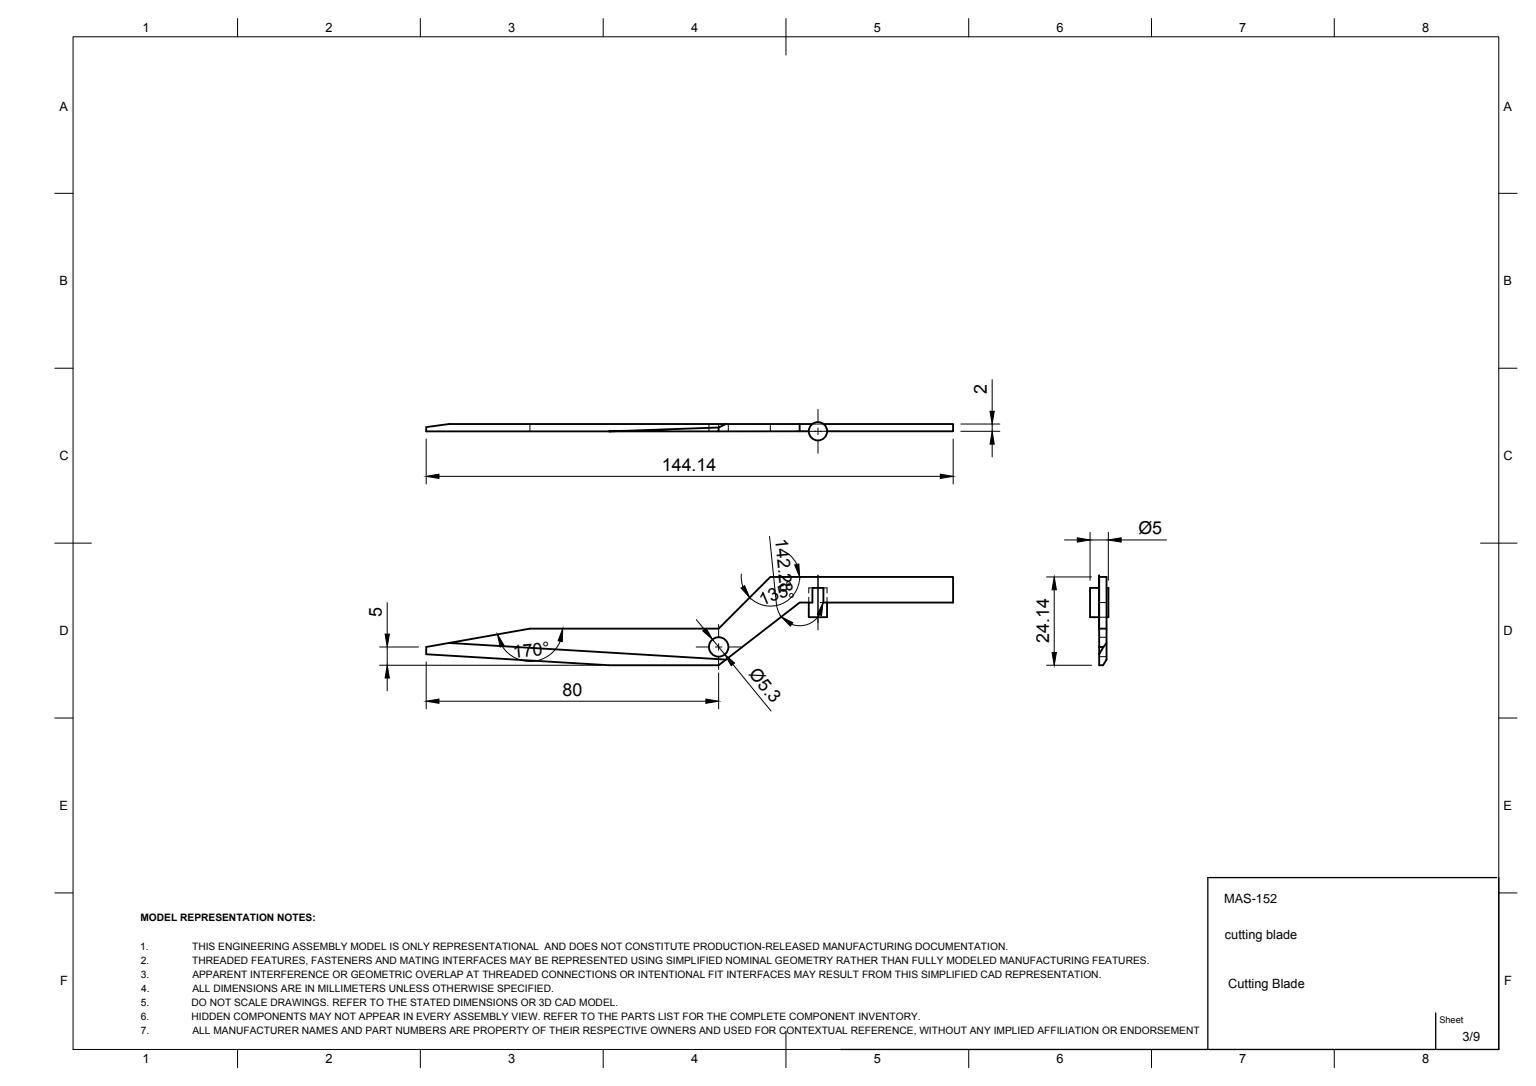
ISO-10303-21;
HEADER;
/* Generated by software containing ST-Developer
 * from STEP Tools, Inc. (www.steptools.com) 
 */

FILE_DESCRIPTION(
/* description */ ('STEP AP214'),
/* implementation_level */ '2;1');

FILE_NAME(
/* name */ 'Cutting Blade.step',
/* time_stamp */ '2026-11-04T19:18:53-08:00',
/* author */ (''),
/* organization */ (''),
/* preprocessor_version */ 'ST-DEVELOPER v20.2',
/* originating_system */ 'Autodesk Translation Framework v15.17.0.0',
/* authorisation */ '');

FILE_SCHEMA (('AUTOMOTIVE_DESIGN { 1 0 10303 214 3 1 1 }'));
ENDSEC;

DATA;
#10=MECHANICAL_DESIGN_GEOMETRIC_PRESENTATION_REPRESENTATION('',(#81),#5942);
#67=SHAPE_REPRESENTATION_RELATIONSHIP('SRR','None',#5978,#74);
#74=ADVANCED_BREP_SHAPE_REPRESENTATION('',(#88),#5938);
#81=STYLED_ITEM('',(#6022),#88);
#88=MANIFOLD_SOLID_BREP('Body1',#928);
#94=FACE_BOUND('',#217,.T.);
#95=FACE_BOUND('',#219,.T.);
#106=PLANE('',#1051);
#107=PLANE('',#1052);
#108=PLANE('',#1053);
#109=PLANE('',#1054);
#110=PLANE('',#1055);
#111=PLANE('',#1056);
#112=PLANE('',#1057);
#113=PLANE('',#1058);
#114=PLANE('',#1059);
#115=PLANE('',#1060);
#116=PLANE('',#1061);
#117=PLANE('',#1062);
#118=PLANE('',#1063);
#119=PLANE('',#1064);
#120=PLANE('',#1065);
#121=PLANE('',#1066);
#154=FACE_OUTER_BOUND('',#210,.T.);
#155=FACE_OUTER_BOUND('',#211,.T.);
#156=FACE_OUTER_BOUND('',#212,.T.);
#157=FACE_OUTER_BOUND('',#213,.T.);
#158=FACE_OUTER_BOUND('',#214,.T.);
#159=FACE_OUTER_BOUND('',#215,.T.);
#160=FACE_OUTER_BOUND('',#216,.T.);
#161=FACE_OUTER_BOUND('',#218,.T.);
#162=FACE_OUTER_BOUND('',#220,.T.);
#163=FACE_OUTER_BOUND('',#221,.T.);
#164=FACE_OUTER_BOUND('',#222,.T.);
#165=FACE_OUTER_BOUND('',#223,.T.);
#166=FACE_OUTER_BOUND('',#224,.T.);
#167=FACE_OUTER_BOUND('',#225,.T.);
#168=FACE_OUTER_BOUND('',#226,.T.);
#169=FACE_OUTER_BOUND('',#227,.T.);
#170=FACE_OUTER_BOUND('',#228,.T.);
#171=FACE_OUTER_BOUND('',#229,.T.);
#210=EDGE_LOOP('',(#682,#683,#684,#685));
#211=EDGE_LOOP('',(#686,#687,#688,#689,#690,#691,#692,#693,#694,#695,#696,
#697));
#212=EDGE_LOOP('',(#698,#699,#700,#701));
#213=EDGE_LOOP('',(#702,#703,#704,#705));
#214=EDGE_LOOP('',(#706,#707,#708));
#215=EDGE_LOOP('',(#709,#710,#711));
#216=EDGE_LOOP('',(#712,#713,#714,#715,#716,#717,#718,#719,#720,#721,#722,
#723));
#217=EDGE_LOOP('',(#724));
#218=EDGE_LOOP('',(#725,#726,#727,#728,#729,#730,#731,#732,#733,#734,#735,
#736,#737,#738));
#219=EDGE_LOOP('',(#739));
#220=EDGE_LOOP('',(#740,#741,#742,#743,#744));
#221=EDGE_LOOP('',(#745,#746,#747,#748));
#222=EDGE_LOOP('',(#749,#750,#751,#752));
#223=EDGE_LOOP('',(#753,#754,#755,#756));
#224=EDGE_LOOP('',(#757,#758,#759,#760));
#225=EDGE_LOOP('',(#761,#762,#763,#764,#765));
#226=EDGE_LOOP('',(#766,#767,#768,#769,#770,#771));
#227=EDGE_LOOP('',(#772,#773));
#228=EDGE_LOOP('',(#774));
#229=EDGE_LOOP('',(#775,#776,#777));
#260=LINE('',#5725,#338);
#261=LINE('',#5731,#339);
#262=LINE('',#5735,#340);
#263=LINE('',#5739,#341);
#264=LINE('',#5743,#342);
#265=LINE('',#5747,#343);
#266=LINE('',#5751,#344);
#267=LINE('',#5753,#345);
#268=LINE('',#5754,#346);
#269=LINE('',#5758,#347);
#270=LINE('',#5760,#348);
#271=LINE('',#5762,#349);
#272=LINE('',#5763,#350);
#273=LINE('',#5767,#351);
#274=LINE('',#5769,#352);
#275=LINE('',#5770,#353);
#276=LINE('',#5774,#354);
#277=LINE('',#5776,#355);
#278=LINE('',#5777,#356);
#279=LINE('',#5779,#357);
#280=LINE('',#5781,#358);
#281=LINE('',#5783,#359);
#282=LINE('',#5784,#360);
#283=LINE('',#5786,#361);
#284=LINE('',#5788,#362);
#285=LINE('',#5790,#363);
#286=LINE('',#5791,#364);
#287=LINE('',#5793,#365);
#288=LINE('',#5795,#366);
#289=LINE('',#5796,#367);
#290=LINE('',#5797,#368);
#291=LINE('',#5798,#369);
#292=LINE('',#5800,#370);
#293=LINE('',#5802,#371);
#294=LINE('',#5803,#372);
#295=LINE('',#5805,#373);
#296=LINE('',#5806,#374);
#297=LINE('',#5808,#375);
#298=LINE('',#5810,#376);
#299=LINE('',#5814,#377);
#338=VECTOR('',#1181,2.65);
#339=VECTOR('',#1188,2.5);
#340=VECTOR('',#1191,1000.);
#341=VECTOR('',#1194,1000.);
#342=VECTOR('',#1197,1000.);
#343=VECTOR('',#1200,1000.);
#344=VECTOR('',#1205,1000.);
#345=VECTOR('',#1206,1000.);
#346=VECTOR('',#1207,1000.);
#347=VECTOR('',#1210,1000.);
#348=VECTOR('',#1211,1000.);
#349=VECTOR('',#1212,1000.);
#350=VECTOR('',#1213,1000.);
#351=VECTOR('',#1216,1000.);
#352=VECTOR('',#1217,1000.);
#353=VECTOR('',#1218,1000.);
#354=VECTOR('',#1221,1000.);
#355=VECTOR('',#1222,1000.);
#356=VECTOR('',#1223,1000.);
#357=VECTOR('',#1226,1000.);
#358=VECTOR('',#1227,1000.);
#359=VECTOR('',#1228,1000.);
#360=VECTOR('',#1229,1000.);
#361=VECTOR('',#1230,1000.);
#362=VECTOR('',#1231,1000.);
#363=VECTOR('',#1232,1000.);
#364=VECTOR('',#1233,1000.);
#365=VECTOR('',#1236,1000.);
#366=VECTOR('',#1237,1000.);
#367=VECTOR('',#1238,1000.);
#368=VECTOR('',#1239,1000.);
#369=VECTOR('',#1240,1000.);
#370=VECTOR('',#1241,1000.);
#371=VECTOR('',#1242,1000.);
#372=VECTOR('',#1243,1000.);
#373=VECTOR('',#1246,1000.);
#374=VECTOR('',#1247,1000.);
#375=VECTOR('',#1250,1000.);
#376=VECTOR('',#1253,1000.);
#377=VECTOR('',#1260,1000.);
#428=CIRCLE('',#1042,2.65);
#429=CIRCLE('',#1043,2.65);
#430=CIRCLE('',#1045,2.5);
#431=CIRCLE('',#1046,2.5);
#432=CIRCLE('',#1047,2.5);
#433=CIRCLE('',#1048,2.5);
#434=CIRCLE('',#1049,2.5);
#435=CIRCLE('',#1050,2.5);
#460=VERTEX_POINT('',#5722);
#461=VERTEX_POINT('',#5724);
#462=VERTEX_POINT('',#5728);
#463=VERTEX_POINT('',#5730);
#464=VERTEX_POINT('',#5732);
#465=VERTEX_POINT('',#5734);
#466=VERTEX_POINT('',#5736);
#467=VERTEX_POINT('',#5738);
#468=VERTEX_POINT('',#5740);
#469=VERTEX_POINT('',#5742);
#470=VERTEX_POINT('',#5744);
#471=VERTEX_POINT('',#5746);
#472=VERTEX_POINT('',#5750);
#473=VERTEX_POINT('',#5752);
#474=VERTEX_POINT('',#5756);
#475=VERTEX_POINT('',#5757);
#476=VERTEX_POINT('',#5759);
#477=VERTEX_POINT('',#5761);
#478=VERTEX_POINT('',#5765);
#479=VERTEX_POINT('',#5766);
#480=VERTEX_POINT('',#5768);
#481=VERTEX_POINT('',#5772);
#482=VERTEX_POINT('',#5773);
#483=VERTEX_POINT('',#5775);
#484=VERTEX_POINT('',#5780);
#485=VERTEX_POINT('',#5782);
#486=VERTEX_POINT('',#5785);
#487=VERTEX_POINT('',#5787);
#488=VERTEX_POINT('',#5789);
#489=VERTEX_POINT('',#5794);
#490=VERTEX_POINT('',#5799);
#491=VERTEX_POINT('',#5801);
#544=EDGE_CURVE('',#460,#460,#428,.T.);
#545=EDGE_CURVE('',#460,#461,#260,.T.);
#546=EDGE_CURVE('',#461,#461,#429,.T.);
#547=EDGE_CURVE('',#462,#462,#430,.T.);
#548=EDGE_CURVE('',#462,#463,#261,.T.);
#549=EDGE_CURVE('',#463,#464,#431,.T.);
#550=EDGE_CURVE('',#464,#465,#262,.T.);
#551=EDGE_CURVE('',#465,#466,#432,.T.);
#552=EDGE_CURVE('',#467,#466,#263,.T.);
#553=EDGE_CURVE('',#467,#468,#433,.T.);
#554=EDGE_CURVE('',#469,#468,#264,.T.);
#555=EDGE_CURVE('',#469,#470,#434,.T.);
#556=EDGE_CURVE('',#470,#471,#265,.T.);
#557=EDGE_CURVE('',#471,#463,#435,.T.);
#558=EDGE_CURVE('',#465,#472,#266,.T.);
#559=EDGE_CURVE('',#472,#473,#267,.T.);
#560=EDGE_CURVE('',#466,#473,#268,.T.);
#561=EDGE_CURVE('',#474,#475,#269,.T.);
#562=EDGE_CURVE('',#475,#476,#270,.T.);
#563=EDGE_CURVE('',#477,#476,#271,.T.);
#564=EDGE_CURVE('',#477,#474,#272,.T.);
#565=EDGE_CURVE('',#478,#479,#273,.T.);
#566=EDGE_CURVE('',#478,#480,#274,.T.);
#567=EDGE_CURVE('',#480,#479,#275,.T.);
#568=EDGE_CURVE('',#481,#482,#276,.T.);
#569=EDGE_CURVE('',#481,#483,#277,.T.);
#570=EDGE_CURVE('',#482,#483,#278,.T.);
#571=EDGE_CURVE('',#467,#468,#279,.T.);
#572=EDGE_CURVE('',#473,#484,#280,.T.);
#573=EDGE_CURVE('',#484,#485,#281,.T.);
#574=EDGE_CURVE('',#485,#477,#282,.T.);
#575=EDGE_CURVE('',#476,#486,#283,.T.);
#576=EDGE_CURVE('',#486,#487,#284,.T.);
#577=EDGE_CURVE('',#487,#488,#285,.T.);
#578=EDGE_CURVE('',#488,#469,#286,.T.);
#579=EDGE_CURVE('',#464,#471,#287,.T.);
#580=EDGE_CURVE('',#489,#470,#288,.T.);
#581=EDGE_CURVE('',#482,#489,#289,.T.);
#582=EDGE_CURVE('',#483,#478,#290,.T.);
#583=EDGE_CURVE('',#479,#475,#291,.T.);
#584=EDGE_CURVE('',#490,#474,#292,.T.);
#585=EDGE_CURVE('',#491,#490,#293,.T.);
#586=EDGE_CURVE('',#472,#491,#294,.T.);
#587=EDGE_CURVE('',#487,#481,#295,.T.);
#588=EDGE_CURVE('',#489,#488,#296,.T.);
#589=EDGE_CURVE('',#490,#485,#297,.T.);
#590=EDGE_CURVE('',#491,#484,#298,.T.);
#591=EDGE_CURVE('',#480,#486,#299,.T.);
#682=ORIENTED_EDGE('',*,*,#544,.T.);
#683=ORIENTED_EDGE('',*,*,#545,.T.);
#684=ORIENTED_EDGE('',*,*,#546,.T.);
#685=ORIENTED_EDGE('',*,*,#545,.F.);
#686=ORIENTED_EDGE('',*,*,#547,.F.);
#687=ORIENTED_EDGE('',*,*,#548,.T.);
#688=ORIENTED_EDGE('',*,*,#549,.T.);
#689=ORIENTED_EDGE('',*,*,#550,.T.);
#690=ORIENTED_EDGE('',*,*,#551,.T.);
#691=ORIENTED_EDGE('',*,*,#552,.F.);
#692=ORIENTED_EDGE('',*,*,#553,.T.);
#693=ORIENTED_EDGE('',*,*,#554,.F.);
#694=ORIENTED_EDGE('',*,*,#555,.T.);
#695=ORIENTED_EDGE('',*,*,#556,.T.);
#696=ORIENTED_EDGE('',*,*,#557,.T.);
#697=ORIENTED_EDGE('',*,*,#548,.F.);
#698=ORIENTED_EDGE('',*,*,#551,.F.);
#699=ORIENTED_EDGE('',*,*,#558,.T.);
#700=ORIENTED_EDGE('',*,*,#559,.T.);
#701=ORIENTED_EDGE('',*,*,#560,.F.);
#702=ORIENTED_EDGE('',*,*,#561,.T.);
#703=ORIENTED_EDGE('',*,*,#562,.T.);
#704=ORIENTED_EDGE('',*,*,#563,.F.);
#705=ORIENTED_EDGE('',*,*,#564,.T.);
#706=ORIENTED_EDGE('',*,*,#565,.F.);
#707=ORIENTED_EDGE('',*,*,#566,.T.);
#708=ORIENTED_EDGE('',*,*,#567,.T.);
#709=ORIENTED_EDGE('',*,*,#568,.F.);
#710=ORIENTED_EDGE('',*,*,#569,.T.);
#711=ORIENTED_EDGE('',*,*,#570,.F.);
#712=ORIENTED_EDGE('',*,*,#571,.F.);
#713=ORIENTED_EDGE('',*,*,#552,.T.);
#714=ORIENTED_EDGE('',*,*,#560,.T.);
#715=ORIENTED_EDGE('',*,*,#572,.T.);
#716=ORIENTED_EDGE('',*,*,#573,.T.);
#717=ORIENTED_EDGE('',*,*,#574,.T.);
#718=ORIENTED_EDGE('',*,*,#563,.T.);
#719=ORIENTED_EDGE('',*,*,#575,.T.);
#720=ORIENTED_EDGE('',*,*,#576,.T.);
#721=ORIENTED_EDGE('',*,*,#577,.T.);
#722=ORIENTED_EDGE('',*,*,#578,.T.);
#723=ORIENTED_EDGE('',*,*,#554,.T.);
#724=ORIENTED_EDGE('',*,*,#546,.F.);
#725=ORIENTED_EDGE('',*,*,#550,.F.);
#726=ORIENTED_EDGE('',*,*,#579,.T.);
#727=ORIENTED_EDGE('',*,*,#556,.F.);
#728=ORIENTED_EDGE('',*,*,#580,.F.);
#729=ORIENTED_EDGE('',*,*,#581,.F.);
#730=ORIENTED_EDGE('',*,*,#570,.T.);
#731=ORIENTED_EDGE('',*,*,#582,.T.);
#732=ORIENTED_EDGE('',*,*,#565,.T.);
#733=ORIENTED_EDGE('',*,*,#583,.T.);
#734=ORIENTED_EDGE('',*,*,#561,.F.);
#735=ORIENTED_EDGE('',*,*,#584,.F.);
#736=ORIENTED_EDGE('',*,*,#585,.F.);
#737=ORIENTED_EDGE('',*,*,#586,.F.);
#738=ORIENTED_EDGE('',*,*,#558,.F.);
#739=ORIENTED_EDGE('',*,*,#544,.F.);
#740=ORIENTED_EDGE('',*,*,#577,.F.);
#741=ORIENTED_EDGE('',*,*,#587,.T.);
#742=ORIENTED_EDGE('',*,*,#568,.T.);
#743=ORIENTED_EDGE('',*,*,#581,.T.);
#744=ORIENTED_EDGE('',*,*,#588,.T.);
#745=ORIENTED_EDGE('',*,*,#574,.F.);
#746=ORIENTED_EDGE('',*,*,#589,.F.);
#747=ORIENTED_EDGE('',*,*,#584,.T.);
#748=ORIENTED_EDGE('',*,*,#564,.F.);
#749=ORIENTED_EDGE('',*,*,#573,.F.);
#750=ORIENTED_EDGE('',*,*,#590,.F.);
#751=ORIENTED_EDGE('',*,*,#585,.T.);
#752=ORIENTED_EDGE('',*,*,#589,.T.);
#753=ORIENTED_EDGE('',*,*,#572,.F.);
#754=ORIENTED_EDGE('',*,*,#559,.F.);
#755=ORIENTED_EDGE('',*,*,#586,.T.);
#756=ORIENTED_EDGE('',*,*,#590,.T.);
#757=ORIENTED_EDGE('',*,*,#555,.F.);
#758=ORIENTED_EDGE('',*,*,#578,.F.);
#759=ORIENTED_EDGE('',*,*,#588,.F.);
#760=ORIENTED_EDGE('',*,*,#580,.T.);
#761=ORIENTED_EDGE('',*,*,#567,.F.);
#762=ORIENTED_EDGE('',*,*,#591,.T.);
#763=ORIENTED_EDGE('',*,*,#575,.F.);
#764=ORIENTED_EDGE('',*,*,#562,.F.);
#765=ORIENTED_EDGE('',*,*,#583,.F.);
#766=ORIENTED_EDGE('',*,*,#566,.F.);
#767=ORIENTED_EDGE('',*,*,#582,.F.);
#768=ORIENTED_EDGE('',*,*,#569,.F.);
#769=ORIENTED_EDGE('',*,*,#587,.F.);
#770=ORIENTED_EDGE('',*,*,#576,.F.);
#771=ORIENTED_EDGE('',*,*,#591,.F.);
#772=ORIENTED_EDGE('',*,*,#553,.F.);
#773=ORIENTED_EDGE('',*,*,#571,.T.);
#774=ORIENTED_EDGE('',*,*,#547,.T.);
#775=ORIENTED_EDGE('',*,*,#579,.F.);
#776=ORIENTED_EDGE('',*,*,#549,.F.);
#777=ORIENTED_EDGE('',*,*,#557,.F.);
#865=CYLINDRICAL_SURFACE('',#1041,2.65);
#866=CYLINDRICAL_SURFACE('',#1044,2.5);
#885=ADVANCED_FACE('',(#154),#865,.F.);
#886=ADVANCED_FACE('',(#155),#866,.T.);
#887=ADVANCED_FACE('',(#156),#106,.T.);
#888=ADVANCED_FACE('',(#157),#107,.F.);
#889=ADVANCED_FACE('',(#158),#108,.T.);
#890=ADVANCED_FACE('',(#159),#109,.T.);
#891=ADVANCED_FACE('',(#160,#94),#110,.F.);
#892=ADVANCED_FACE('',(#161,#95),#111,.T.);
#893=ADVANCED_FACE('',(#162),#112,.T.);
#894=ADVANCED_FACE('',(#163),#113,.T.);
#895=ADVANCED_FACE('',(#164),#114,.T.);
#896=ADVANCED_FACE('',(#165),#115,.T.);
#897=ADVANCED_FACE('',(#166),#116,.T.);
#898=ADVANCED_FACE('',(#167),#117,.T.);
#899=ADVANCED_FACE('',(#168),#118,.F.);
#900=ADVANCED_FACE('',(#169),#119,.F.);
#901=ADVANCED_FACE('',(#170),#120,.T.);
#902=ADVANCED_FACE('',(#171),#121,.F.);
#928=CLOSED_SHELL('',(#885,#886,#887,#888,#889,#890,#891,#892,#893,#894,
#895,#896,#897,#898,#899,#900,#901,#902));
#1040=AXIS2_PLACEMENT_3D('',#5720,#1175,#1176);
#1041=AXIS2_PLACEMENT_3D('',#5721,#1177,#1178);
#1042=AXIS2_PLACEMENT_3D('',#5723,#1179,#1180);
#1043=AXIS2_PLACEMENT_3D('',#5726,#1182,#1183);
#1044=AXIS2_PLACEMENT_3D('',#5727,#1184,#1185);
#1045=AXIS2_PLACEMENT_3D('',#5729,#1186,#1187);
#1046=AXIS2_PLACEMENT_3D('',#5733,#1189,#1190);
#1047=AXIS2_PLACEMENT_3D('',#5737,#1192,#1193);
#1048=AXIS2_PLACEMENT_3D('',#5741,#1195,#1196);
#1049=AXIS2_PLACEMENT_3D('',#5745,#1198,#1199);
#1050=AXIS2_PLACEMENT_3D('',#5748,#1201,#1202);
#1051=AXIS2_PLACEMENT_3D('',#5749,#1203,#1204);
#1052=AXIS2_PLACEMENT_3D('',#5755,#1208,#1209);
#1053=AXIS2_PLACEMENT_3D('',#5764,#1214,#1215);
#1054=AXIS2_PLACEMENT_3D('',#5771,#1219,#1220);
#1055=AXIS2_PLACEMENT_3D('',#5778,#1224,#1225);
#1056=AXIS2_PLACEMENT_3D('',#5792,#1234,#1235);
#1057=AXIS2_PLACEMENT_3D('',#5804,#1244,#1245);
#1058=AXIS2_PLACEMENT_3D('',#5807,#1248,#1249);
#1059=AXIS2_PLACEMENT_3D('',#5809,#1251,#1252);
#1060=AXIS2_PLACEMENT_3D('',#5811,#1254,#1255);
#1061=AXIS2_PLACEMENT_3D('',#5812,#1256,#1257);
#1062=AXIS2_PLACEMENT_3D('',#5813,#1258,#1259);
#1063=AXIS2_PLACEMENT_3D('',#5815,#1261,#1262);
#1064=AXIS2_PLACEMENT_3D('',#5816,#1263,#1264);
#1065=AXIS2_PLACEMENT_3D('',#5817,#1265,#1266);
#1066=AXIS2_PLACEMENT_3D('',#5818,#1267,#1268);
#1175=DIRECTION('axis',(0.,0.,1.));
#1176=DIRECTION('refdir',(1.,0.,0.));
#1177=DIRECTION('center_axis',(0.,0.,1.));
#1178=DIRECTION('ref_axis',(1.,0.,0.));
#1179=DIRECTION('center_axis',(0.,0.,-1.));
#1180=DIRECTION('ref_axis',(-1.,0.,0.));
#1181=DIRECTION('',(0.,0.,1.));
#1182=DIRECTION('center_axis',(0.,0.,1.));
#1183=DIRECTION('ref_axis',(1.,0.,0.));
#1184=DIRECTION('center_axis',(-1.,0.,0.));
#1185=DIRECTION('ref_axis',(0.,0.,1.));
#1186=DIRECTION('center_axis',(-1.,0.,0.));
#1187=DIRECTION('ref_axis',(0.,0.,1.));
#1188=DIRECTION('',(1.,0.,0.));
#1189=DIRECTION('center_axis',(-1.,0.,0.));
#1190=DIRECTION('ref_axis',(0.,0.,1.));
#1191=DIRECTION('',(-1.,0.,0.));
#1192=DIRECTION('center_axis',(-1.,-1.51313062618285E-16,0.));
#1193=DIRECTION('ref_axis',(1.51313062618285E-16,-1.,0.));
#1194=DIRECTION('',(-1.,0.,0.));
#1195=DIRECTION('center_axis',(-1.,0.,0.));
#1196=DIRECTION('ref_axis',(0.,0.,1.));
#1197=DIRECTION('',(1.,0.,0.));
#1198=DIRECTION('center_axis',(-1.,-1.51313062618285E-16,0.));
#1199=DIRECTION('ref_axis',(1.51313062618285E-16,-1.,0.));
#1200=DIRECTION('',(1.,0.,0.));
#1201=DIRECTION('center_axis',(-1.,0.,0.));
#1202=DIRECTION('ref_axis',(0.,0.,1.));
#1203=DIRECTION('center_axis',(-1.,-1.51313062618285E-16,0.));
#1204=DIRECTION('ref_axis',(1.51313062618285E-16,-1.,0.));
#1205=DIRECTION('',(1.51313062618285E-16,-1.,0.));
#1206=DIRECTION('',(0.,0.,1.));
#1207=DIRECTION('',(1.51313062618285E-16,-1.,0.));
#1208=DIRECTION('center_axis',(-1.,0.,0.));
#1209=DIRECTION('ref_axis',(0.,0.,1.));
#1210=DIRECTION('',(0.,1.,0.));
#1211=DIRECTION('',(0.,0.,1.));
#1212=DIRECTION('',(0.,1.,0.));
#1213=DIRECTION('',(0.,0.,-1.));
#1214=DIRECTION('center_axis',(0.,1.,0.));
#1215=DIRECTION('ref_axis',(0.,0.,1.));
#1216=DIRECTION('',(1.,0.,0.));
#1217=DIRECTION('',(0.866413978654257,0.,0.499326363806779));
#1218=DIRECTION('',(0.,0.,-1.));
#1219=DIRECTION('center_axis',(-1.,0.,0.));
#1220=DIRECTION('ref_axis',(0.,0.,1.));
#1221=DIRECTION('',(0.,0.,-1.));
#1222=DIRECTION('',(0.,0.999402687851137,-0.0345581758188068));
#1223=DIRECTION('',(0.,1.,0.));
#1224=DIRECTION('center_axis',(0.,0.,-1.));
#1225=DIRECTION('ref_axis',(-1.,0.,0.));
#1226=DIRECTION('',(0.,1.,0.));
#1227=DIRECTION('',(1.,0.,0.));
#1228=DIRECTION('',(-6.93889390390723E-17,1.,0.));
#1229=DIRECTION('',(-0.707106781186544,0.707106781186551,0.));
#1230=DIRECTION('',(-0.17364817766693,0.984807753012208,0.));
#1231=DIRECTION('',(-0.0598922907279467,-0.998204845465779,0.));
#1232=DIRECTION('',(0.611809881784581,-0.791004847362351,0.));
#1233=DIRECTION('',(1.51313062618285E-16,-1.,0.));
#1234=DIRECTION('center_axis',(0.,0.,-1.));
#1235=DIRECTION('ref_axis',(-1.,0.,0.));
#1236=DIRECTION('',(0.,1.,0.));
#1237=DIRECTION('',(1.51313062618285E-16,-1.,0.));
#1238=DIRECTION('',(0.611809881784581,-0.791004847362351,0.));
#1239=DIRECTION('',(0.0598922907279467,0.998204845465779,0.));
#1240=DIRECTION('',(0.17364817766693,-0.984807753012208,0.));
#1241=DIRECTION('',(-0.707106781186544,0.707106781186551,0.));
#1242=DIRECTION('',(-6.93889390390723E-17,1.,0.));
#1243=DIRECTION('',(1.,0.,0.));
#1244=DIRECTION('center_axis',(-0.791004847362351,-0.611809881784581,0.));
#1245=DIRECTION('ref_axis',(0.611809881784581,-0.791004847362351,0.));
#1246=DIRECTION('',(-0.571919987099744,0.739431473025142,-0.355174077116697));
#1247=DIRECTION('',(0.,0.,1.));
#1248=DIRECTION('center_axis',(0.707106781186551,0.707106781186544,0.));
#1249=DIRECTION('ref_axis',(-0.707106781186544,0.707106781186551,0.));
#1250=DIRECTION('',(0.,0.,1.));
#1251=DIRECTION('center_axis',(1.,6.93889390390723E-17,0.));
#1252=DIRECTION('ref_axis',(-6.93889390390723E-17,1.,0.));
#1253=DIRECTION('',(0.,0.,1.));
#1254=DIRECTION('center_axis',(0.,-1.,0.));
#1255=DIRECTION('ref_axis',(0.,0.,-1.));
#1256=DIRECTION('center_axis',(-1.,-1.51313062618285E-16,0.));
#1257=DIRECTION('ref_axis',(1.51313062618285E-16,-1.,0.));
#1258=DIRECTION('center_axis',(0.984807753012208,0.17364817766693,0.));
#1259=DIRECTION('ref_axis',(0.,0.,1.));
#1260=DIRECTION('',(0.172106918435043,-0.976066837551089,0.132938847820377));
#1261=DIRECTION('center_axis',(0.499102422732889,-0.0299461453639734,-0.866025403784439));
#1262=DIRECTION('ref_axis',(-0.0598922907279467,-0.998204845465779,1.0301470331017E-18));
#1263=DIRECTION('center_axis',(-1.,0.,0.));
#1264=DIRECTION('ref_axis',(0.,0.,1.));
#1265=DIRECTION('center_axis',(-1.,0.,0.));
#1266=DIRECTION('ref_axis',(0.,0.,1.));
#1267=DIRECTION('center_axis',(-1.,0.,0.));
#1268=DIRECTION('ref_axis',(0.,0.,1.));
#5720=CARTESIAN_POINT('',(0.,0.,0.));
#5721=CARTESIAN_POINT('Origin',(0.,0.,2.));
#5722=CARTESIAN_POINT('',(-2.65,-3.24531401774049E-16,0.));
#5723=CARTESIAN_POINT('Origin',(0.,0.,0.));
#5724=CARTESIAN_POINT('',(-2.65,-3.24531401774049E-16,2.));
#5725=CARTESIAN_POINT('',(-2.65,-3.24531401774049E-16,2.));
#5726=CARTESIAN_POINT('Origin',(0.,0.,2.));
#5727=CARTESIAN_POINT('Origin',(16.1421356237309,-27.1629509039023,0.));
#5728=CARTESIAN_POINT('',(8.14213562373088,-27.1629509039023,-2.5));
#5729=CARTESIAN_POINT('Origin',(8.14213562373088,-27.1629509039023,0.));
#5730=CARTESIAN_POINT('',(16.1421356237309,-27.1629509039023,-2.5));
#5731=CARTESIAN_POINT('',(16.1421356237309,-27.1629509039023,-2.5));
#5732=CARTESIAN_POINT('',(16.1421356237309,-29.6629509039023,0.));
#5733=CARTESIAN_POINT('Origin',(16.1421356237309,-27.1629509039023,0.));
#5734=CARTESIAN_POINT('',(12.1421356237309,-29.6629509039023,0.));
#5735=CARTESIAN_POINT('',(16.1421356237309,-29.6629509039023,0.));
#5736=CARTESIAN_POINT('',(12.1421356237309,-28.6629509039023,2.));
#5737=CARTESIAN_POINT('Origin',(12.1421356237309,-27.1629509039023,0.));
#5738=CARTESIAN_POINT('',(16.1421356237309,-28.6629509039023,2.));
#5739=CARTESIAN_POINT('',(16.1421356237309,-28.6629509039023,2.));
#5740=CARTESIAN_POINT('',(16.1421356237309,-25.6629509039023,2.));
#5741=CARTESIAN_POINT('Origin',(16.1421356237309,-27.1629509039023,0.));
#5742=CARTESIAN_POINT('',(12.1421356237309,-25.6629509039023,2.));
#5743=CARTESIAN_POINT('',(16.1421356237309,-25.6629509039023,2.));
#5744=CARTESIAN_POINT('',(12.1421356237309,-24.6629509039023,0.));
#5745=CARTESIAN_POINT('Origin',(12.1421356237309,-27.1629509039023,0.));
#5746=CARTESIAN_POINT('',(16.1421356237309,-24.6629509039023,0.));
#5747=CARTESIAN_POINT('',(16.1421356237309,-24.6629509039023,0.));
#5748=CARTESIAN_POINT('Origin',(16.1421356237309,-27.1629509039023,0.));
#5749=CARTESIAN_POINT('Origin',(12.1421356237309,-18.2842712474619,0.));
#5750=CARTESIAN_POINT('',(12.1421356237309,-64.142135623731,0.));
#5751=CARTESIAN_POINT('',(12.1421356237309,-18.2842712474619,0.));
#5752=CARTESIAN_POINT('',(12.1421356237309,-64.142135623731,2.));
#5753=CARTESIAN_POINT('',(12.1421356237309,-64.142135623731,0.));
#5754=CARTESIAN_POINT('',(12.1421356237309,-18.2842712474619,2.));
#5755=CARTESIAN_POINT('Origin',(5.,0.,2.));
#5756=CARTESIAN_POINT('',(5.,0.,0.));
#5757=CARTESIAN_POINT('',(5.,51.6435909019114,0.));
#5758=CARTESIAN_POINT('',(5.,0.,0.));
#5759=CARTESIAN_POINT('',(5.,51.6435909019114,2.));
#5760=CARTESIAN_POINT('',(5.,51.6435909019114,2.));
#5761=CARTESIAN_POINT('',(5.,0.,2.));
#5762=CARTESIAN_POINT('',(5.,0.,2.));
#5763=CARTESIAN_POINT('',(5.,0.,2.));
#5764=CARTESIAN_POINT('Origin',(-5.,80.,2.));
#5765=CARTESIAN_POINT('',(-2.,80.,0.));
#5766=CARTESIAN_POINT('',(-4.33680868994202E-15,80.,0.));
#5767=CARTESIAN_POINT('',(-5.,80.,0.));
#5768=CARTESIAN_POINT('',(-4.33680868994202E-15,80.,1.15262767247211));
#5769=CARTESIAN_POINT('',(-3.38677286419691,80.,-0.799216389353386));
#5770=CARTESIAN_POINT('',(-4.33680868994202E-15,80.,0.));
#5771=CARTESIAN_POINT('Origin',(-5.,0.,2.));
#5772=CARTESIAN_POINT('',(-5.,0.,1.0373649052249));
#5773=CARTESIAN_POINT('',(-5.,0.,0.));
#5774=CARTESIAN_POINT('',(-5.,0.,2.));
#5775=CARTESIAN_POINT('',(-5.,30.,0.));
#5776=CARTESIAN_POINT('',(-5.,-0.0332470421233885,1.03851454904828));
#5777=CARTESIAN_POINT('',(-5.,0.,0.));
#5778=CARTESIAN_POINT('Origin',(0.,0.,2.));
#5779=CARTESIAN_POINT('',(16.1421356237309,0.,2.));
#5780=CARTESIAN_POINT('',(19.1421356237309,-64.142135623731,2.));
#5781=CARTESIAN_POINT('',(9.14213562373088,-64.142135623731,2.));
#5782=CARTESIAN_POINT('',(19.1421356237309,-14.142135623731,2.));
#5783=CARTESIAN_POINT('',(19.1421356237309,-14.142135623731,2.));
#5784=CARTESIAN_POINT('',(5.,0.,2.));
#5785=CARTESIAN_POINT('',(1.09703553512821,73.7784023141528,2.));
#5786=CARTESIAN_POINT('',(-4.33680868994202E-15,80.,2.));
#5787=CARTESIAN_POINT('',(-3.44991431960659,-2.00409526476049,2.));
#5788=CARTESIAN_POINT('',(-1.54211698258366,29.792527018955,2.));
#5789=CARTESIAN_POINT('',(12.1421356237309,-22.1629509039023,2.));
#5790=CARTESIAN_POINT('',(-5.,0.,2.));
#5791=CARTESIAN_POINT('',(12.1421356237309,-18.2842712474619,2.));
#5792=CARTESIAN_POINT('Origin',(0.,0.,0.));
#5793=CARTESIAN_POINT('',(16.1421356237309,0.,0.));
#5794=CARTESIAN_POINT('',(12.1421356237309,-22.1629509039023,0.));
#5795=CARTESIAN_POINT('',(12.1421356237309,-18.2842712474619,0.));
#5796=CARTESIAN_POINT('',(-5.,0.,0.));
#5797=CARTESIAN_POINT('',(-6.77560781187724,0.406536468712635,0.));
#5798=CARTESIAN_POINT('',(13.6808057330267,2.41229516856365,0.));
#5799=CARTESIAN_POINT('',(19.1421356237309,-14.142135623731,0.));
#5800=CARTESIAN_POINT('',(5.,0.,0.));
#5801=CARTESIAN_POINT('',(19.1421356237309,-64.142135623731,0.));
#5802=CARTESIAN_POINT('',(19.1421356237309,-14.142135623731,0.));
#5803=CARTESIAN_POINT('',(9.14213562373088,-64.142135623731,0.));
#5804=CARTESIAN_POINT('Origin',(-5.,0.,0.));
#5805=CARTESIAN_POINT('',(-5.21072112990534,0.272439919915319,0.906502748749744));
#5806=CARTESIAN_POINT('',(12.1421356237309,-22.1629509039023,0.));
#5807=CARTESIAN_POINT('Origin',(5.,0.,0.));
#5808=CARTESIAN_POINT('',(19.1421356237309,-14.142135623731,0.));
#5809=CARTESIAN_POINT('Origin',(19.1421356237309,-14.142135623731,0.));
#5810=CARTESIAN_POINT('',(19.1421356237309,-64.142135623731,0.));
#5811=CARTESIAN_POINT('Origin',(9.14213562373088,-64.142135623731,0.));
#5812=CARTESIAN_POINT('Origin',(12.1421356237309,-18.2842712474619,0.));
#5813=CARTESIAN_POINT('Origin',(-4.33680868994202E-15,80.,2.));
#5814=CARTESIAN_POINT('',(0.019387620776991,79.8900473387618,1.16760306097774));
#5815=CARTESIAN_POINT('Origin',(-3.3177247944609,0.199063487667654,2.));
#5816=CARTESIAN_POINT('Origin',(16.1421356237309,-27.1629509039023,0.));
#5817=CARTESIAN_POINT('Origin',(8.14213562373088,-27.1629509039023,0.));
#5818=CARTESIAN_POINT('Origin',(16.1421356237309,-27.1629509039023,0.));
#5929=UNCERTAINTY_MEASURE_WITH_UNIT(LENGTH_MEASURE(0.01),#5943,
'DISTANCE_ACCURACY_VALUE',
'Maximum model space distance between geometric entities at asserted c
onnectivities');
#5933=UNCERTAINTY_MEASURE_WITH_UNIT(LENGTH_MEASURE(0.01),#5943,
'DISTANCE_ACCURACY_VALUE',
'Maximum model space distance between geometric entities at asserted c
onnectivities');
#5938=(
GEOMETRIC_REPRESENTATION_CONTEXT(3)
GLOBAL_UNCERTAINTY_ASSIGNED_CONTEXT((#5929))
GLOBAL_UNIT_ASSIGNED_CONTEXT((#5943,#5945,#5946))
REPRESENTATION_CONTEXT('','3D')
);
#5942=(
GEOMETRIC_REPRESENTATION_CONTEXT(3)
GLOBAL_UNCERTAINTY_ASSIGNED_CONTEXT((#5933))
GLOBAL_UNIT_ASSIGNED_CONTEXT((#5943,#5945,#5946))
REPRESENTATION_CONTEXT('','3D')
);
#5943=(
LENGTH_UNIT()
NAMED_UNIT(*)
SI_UNIT(.MILLI.,.METRE.)
);
#5945=(
NAMED_UNIT(*)
PLANE_ANGLE_UNIT()
SI_UNIT($,.RADIAN.)
);
#5946=(
NAMED_UNIT(*)
SI_UNIT($,.STERADIAN.)
SOLID_ANGLE_UNIT()
);
#5951=SHAPE_DEFINITION_REPRESENTATION(#5959,#5978);
#5959=PRODUCT_DEFINITION_SHAPE('',$,#5987);
#5978=SHAPE_REPRESENTATION('',(#1040),#5938);
#5982=PRODUCT_DEFINITION_CONTEXT('part definition',#6008,'design');
#5987=PRODUCT_DEFINITION('Cutting Blade','Cutting Blade',#5995,#5982);
#5995=PRODUCT_DEFINITION_FORMATION('',$,#6014);
#6008=APPLICATION_CONTEXT(
'Core Data for Automotive Mechanical Design Process');
#6009=PRODUCT_CONTEXT('part definition',#6008,'mechanical');
#6014=PRODUCT('Cutting Blade','Cutting Blade',$,(#6009));
#6022=PRESENTATION_STYLE_ASSIGNMENT((#6028));
#6028=SURFACE_STYLE_USAGE(.BOTH.,#6034);
#6034=SURFACE_SIDE_STYLE('',(#6040));
#6040=SURFACE_STYLE_FILL_AREA(#6046);
#6046=FILL_AREA_STYLE('Opaque(97,158,199)',(#6052));
#6052=FILL_AREA_STYLE_COLOUR('Opaque(97,158,199)',#6058);
#6058=COLOUR_RGB('Opaque(97,158,199)',0.380392156862745,0.619607843137255,
0.780392156862745);
ENDSEC;
END-ISO-10303-21;
